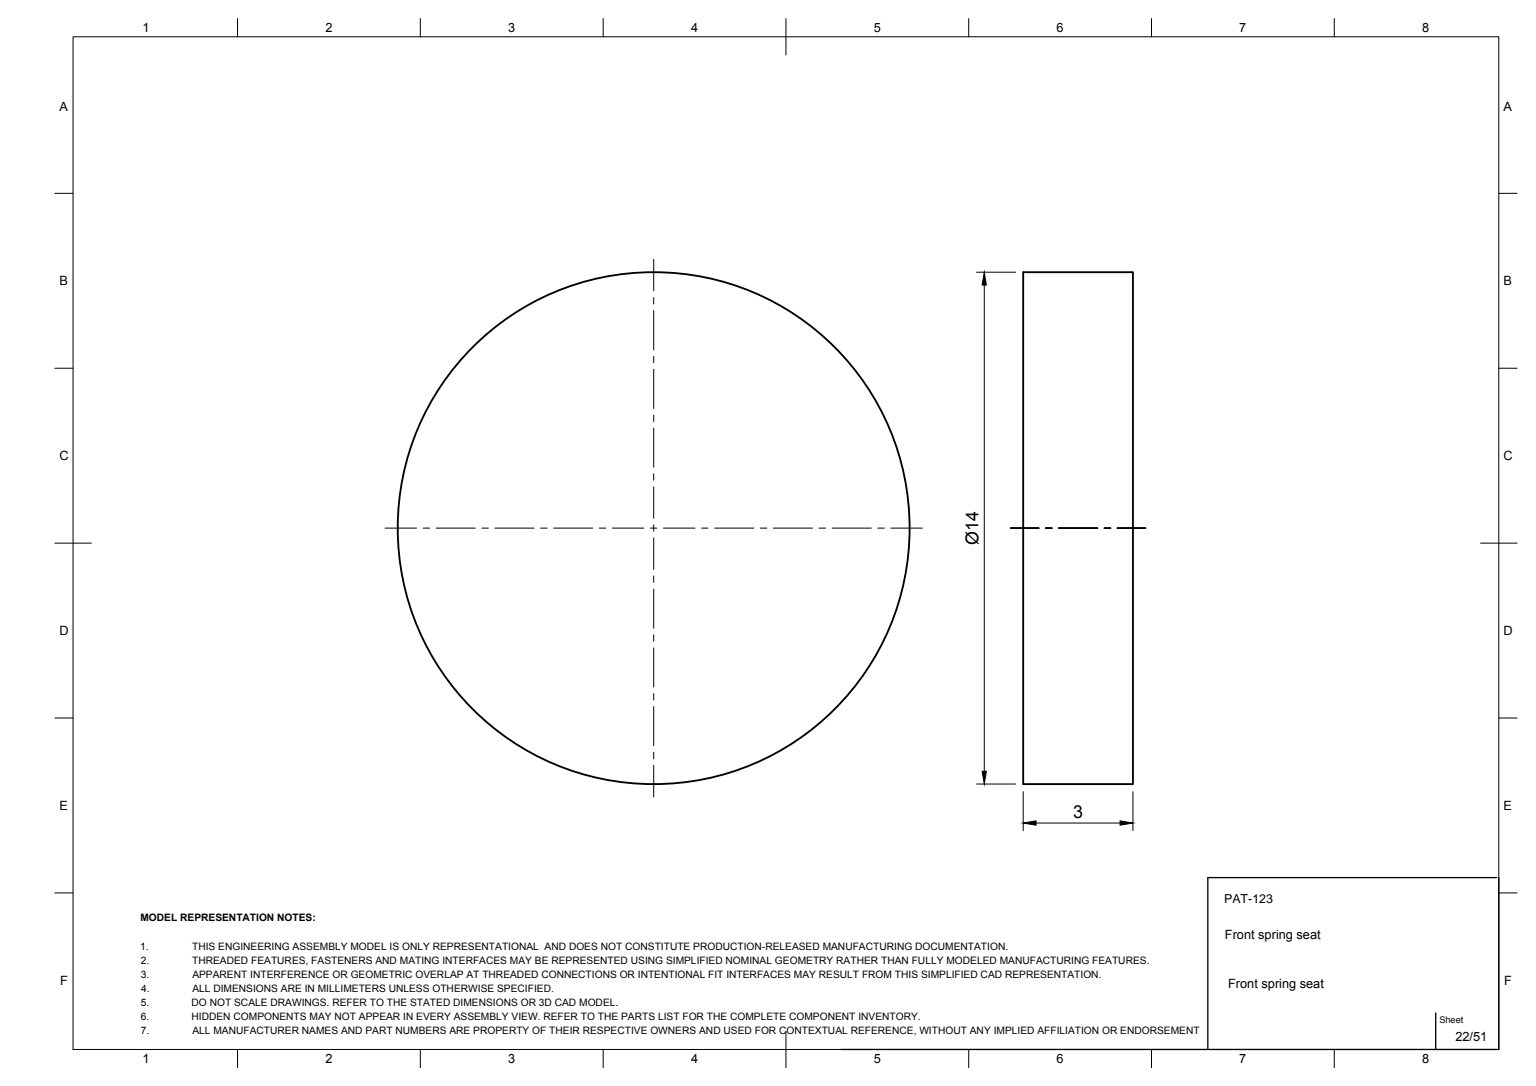
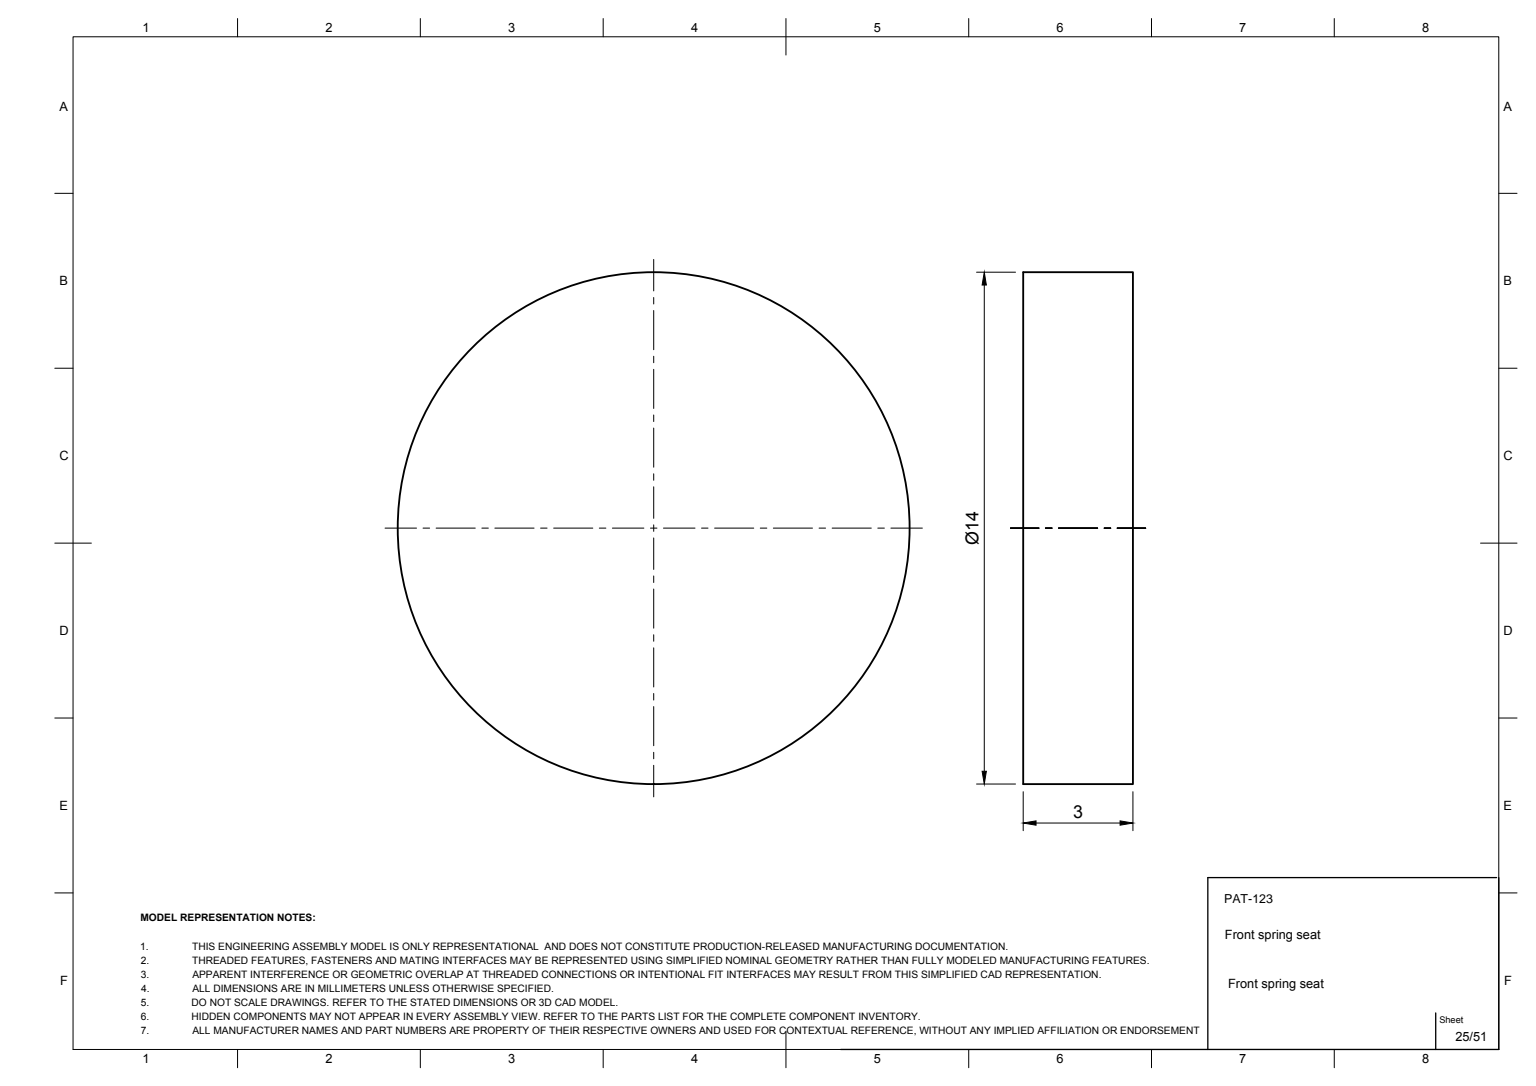
ISO-10303-21;
HEADER;
/* Generated by software containing ST-Developer
 * from STEP Tools, Inc. (www.steptools.com) 
 */

FILE_DESCRIPTION(
/* description */ ('Worm-less right-angle friction wheel drive'),
/* implementation_level */ '2;1');

FILE_NAME(
/* name */ 'Front spring seat.step',
/* time_stamp */ '2026-10-28T03:22:36-07:00',
/* author */ (''),
/* organization */ (''),
/* preprocessor_version */ 'ST-DEVELOPER v20.2',
/* originating_system */ 'Autodesk Translation Framework v15.17.0.0',
/* authorisation */ '');

FILE_SCHEMA (('AUTOMOTIVE_DESIGN { 1 0 10303 214 3 1 1 }'));
ENDSEC;

DATA;
#10=MECHANICAL_DESIGN_GEOMETRIC_PRESENTATION_REPRESENTATION('',(#628),#17046);
#534=SHAPE_REPRESENTATION_RELATIONSHIP('SRR','None',#17277,#581);
#581=ADVANCED_BREP_SHAPE_REPRESENTATION('',(#682),#17013);
#628=STYLED_ITEM('',(#17591),#682);
#682=MANIFOLD_SOLID_BREP('Body1',#8183);
#1056=PLANE('',#9205);
#1057=PLANE('',#9206);
#1424=FACE_OUTER_BOUND('',#2080,.T.);
#1425=FACE_OUTER_BOUND('',#2081,.T.);
#1426=FACE_OUTER_BOUND('',#2082,.T.);
#2080=EDGE_LOOP('',(#6566,#6567,#6568,#6569));
#2081=EDGE_LOOP('',(#6570));
#2082=EDGE_LOOP('',(#6571));
#2669=LINE('',#13475,#3209);
#3209=VECTOR('',#10989,0.7);
#3681=CIRCLE('',#9203,0.7);
#3682=CIRCLE('',#9204,0.7);
#4213=VERTEX_POINT('',#13472);
#4214=VERTEX_POINT('',#13474);
#5052=EDGE_CURVE('',#4213,#4213,#3681,.T.);
#5053=EDGE_CURVE('',#4213,#4214,#2669,.T.);
#5054=EDGE_CURVE('',#4214,#4214,#3682,.T.);
#6566=ORIENTED_EDGE('',*,*,#5052,.F.);
#6567=ORIENTED_EDGE('',*,*,#5053,.T.);
#6568=ORIENTED_EDGE('',*,*,#5054,.T.);
#6569=ORIENTED_EDGE('',*,*,#5053,.F.);
#6570=ORIENTED_EDGE('',*,*,#5052,.T.);
#6571=ORIENTED_EDGE('',*,*,#5054,.F.);
#7642=CYLINDRICAL_SURFACE('',#9202,0.7);
#7916=ADVANCED_FACE('',(#1424),#7642,.T.);
#7917=ADVANCED_FACE('',(#1425),#1056,.T.);
#7918=ADVANCED_FACE('',(#1426),#1057,.F.);
#8183=CLOSED_SHELL('',(#7916,#7917,#7918));
#9201=AXIS2_PLACEMENT_3D('',#13470,#10983,#10984);
#9202=AXIS2_PLACEMENT_3D('',#13471,#10985,#10986);
#9203=AXIS2_PLACEMENT_3D('',#13473,#10987,#10988);
#9204=AXIS2_PLACEMENT_3D('',#13476,#10990,#10991);
#9205=AXIS2_PLACEMENT_3D('',#13477,#10992,#10993);
#9206=AXIS2_PLACEMENT_3D('',#13478,#10994,#10995);
#10983=DIRECTION('axis',(0.,0.,1.));
#10984=DIRECTION('refdir',(1.,0.,0.));
#10985=DIRECTION('center_axis',(0.,1.,0.));
#10986=DIRECTION('ref_axis',(1.,0.,0.));
#10987=DIRECTION('center_axis',(0.,1.,0.));
#10988=DIRECTION('ref_axis',(1.,0.,0.));
#10989=DIRECTION('',(0.,-1.,0.));
#10990=DIRECTION('center_axis',(0.,1.,0.));
#10991=DIRECTION('ref_axis',(1.,0.,0.));
#10992=DIRECTION('center_axis',(0.,1.,0.));
#10993=DIRECTION('ref_axis',(1.,0.,0.));
#10994=DIRECTION('center_axis',(0.,1.,0.));
#10995=DIRECTION('ref_axis',(1.,0.,0.));
#13470=CARTESIAN_POINT('',(0.,0.,0.));
#13471=CARTESIAN_POINT('Origin',(-0.3,5.4,4.));
#13472=CARTESIAN_POINT('',(-1.,5.7,4.));
#13473=CARTESIAN_POINT('Origin',(-0.3,5.7,4.));
#13474=CARTESIAN_POINT('',(-1.,5.4,4.));
#13475=CARTESIAN_POINT('',(-1.,5.4,4.));
#13476=CARTESIAN_POINT('Origin',(-0.3,5.4,4.));
#13477=CARTESIAN_POINT('Origin',(-0.3,5.7,4.));
#13478=CARTESIAN_POINT('Origin',(-0.3,5.4,4.));
#16960=UNCERTAINTY_MEASURE_WITH_UNIT(LENGTH_MEASURE(0.001),#17047,
'DISTANCE_ACCURACY_VALUE',
'Maximum model space distance between geometric entities at asserted c
onnectivities');
#16993=UNCERTAINTY_MEASURE_WITH_UNIT(LENGTH_MEASURE(0.001),#17047,
'DISTANCE_ACCURACY_VALUE',
'Maximum model space distance between geometric entities at asserted c
onnectivities');
#17013=(
GEOMETRIC_REPRESENTATION_CONTEXT(3)
GLOBAL_UNCERTAINTY_ASSIGNED_CONTEXT((#16960))
GLOBAL_UNIT_ASSIGNED_CONTEXT((#17047,#17049,#17050))
REPRESENTATION_CONTEXT('','3D')
);
#17046=(
GEOMETRIC_REPRESENTATION_CONTEXT(3)
GLOBAL_UNCERTAINTY_ASSIGNED_CONTEXT((#16993))
GLOBAL_UNIT_ASSIGNED_CONTEXT((#17047,#17049,#17050))
REPRESENTATION_CONTEXT('','3D')
);
#17047=(
LENGTH_UNIT()
NAMED_UNIT(*)
SI_UNIT(.CENTI.,.METRE.)
);
#17049=(
NAMED_UNIT(*)
PLANE_ANGLE_UNIT()
SI_UNIT($,.RADIAN.)
);
#17050=(
NAMED_UNIT(*)
SI_UNIT($,.STERADIAN.)
SOLID_ANGLE_UNIT()
);
#17070=SHAPE_DEFINITION_REPRESENTATION(#17122,#17277);
#17122=PRODUCT_DEFINITION_SHAPE('',$,#17330);
#17277=SHAPE_REPRESENTATION('',(#9201),#17013);
#17310=PRODUCT_DEFINITION_CONTEXT('part definition',#17468,'design');
#17330=PRODUCT_DEFINITION('Front spring seat','Front spring seat',#17382,
#17310);
#17382=PRODUCT_DEFINITION_FORMATION('',$,#17489);
#17468=APPLICATION_CONTEXT(
'Core Data for Automotive Mechanical Design Process');
#17469=PRODUCT_CONTEXT('part definition',#17468,'mechanical');
#17489=PRODUCT('Front spring seat','Front spring seat',
'Front spring seat',(#17469));
#17585=COLOUR_RGB('Grey',0.48,0.52,0.57);
#17586=FILL_AREA_STYLE_COLOUR('',#17585);
#17587=FILL_AREA_STYLE('',(#17586));
#17588=SURFACE_STYLE_FILL_AREA(#17587);
#17589=SURFACE_SIDE_STYLE('',(#17588));
#17590=SURFACE_STYLE_USAGE(.BOTH.,#17589);
#17591=PRESENTATION_STYLE_ASSIGNMENT((#17590));
ENDSEC;
END-ISO-10303-21;
